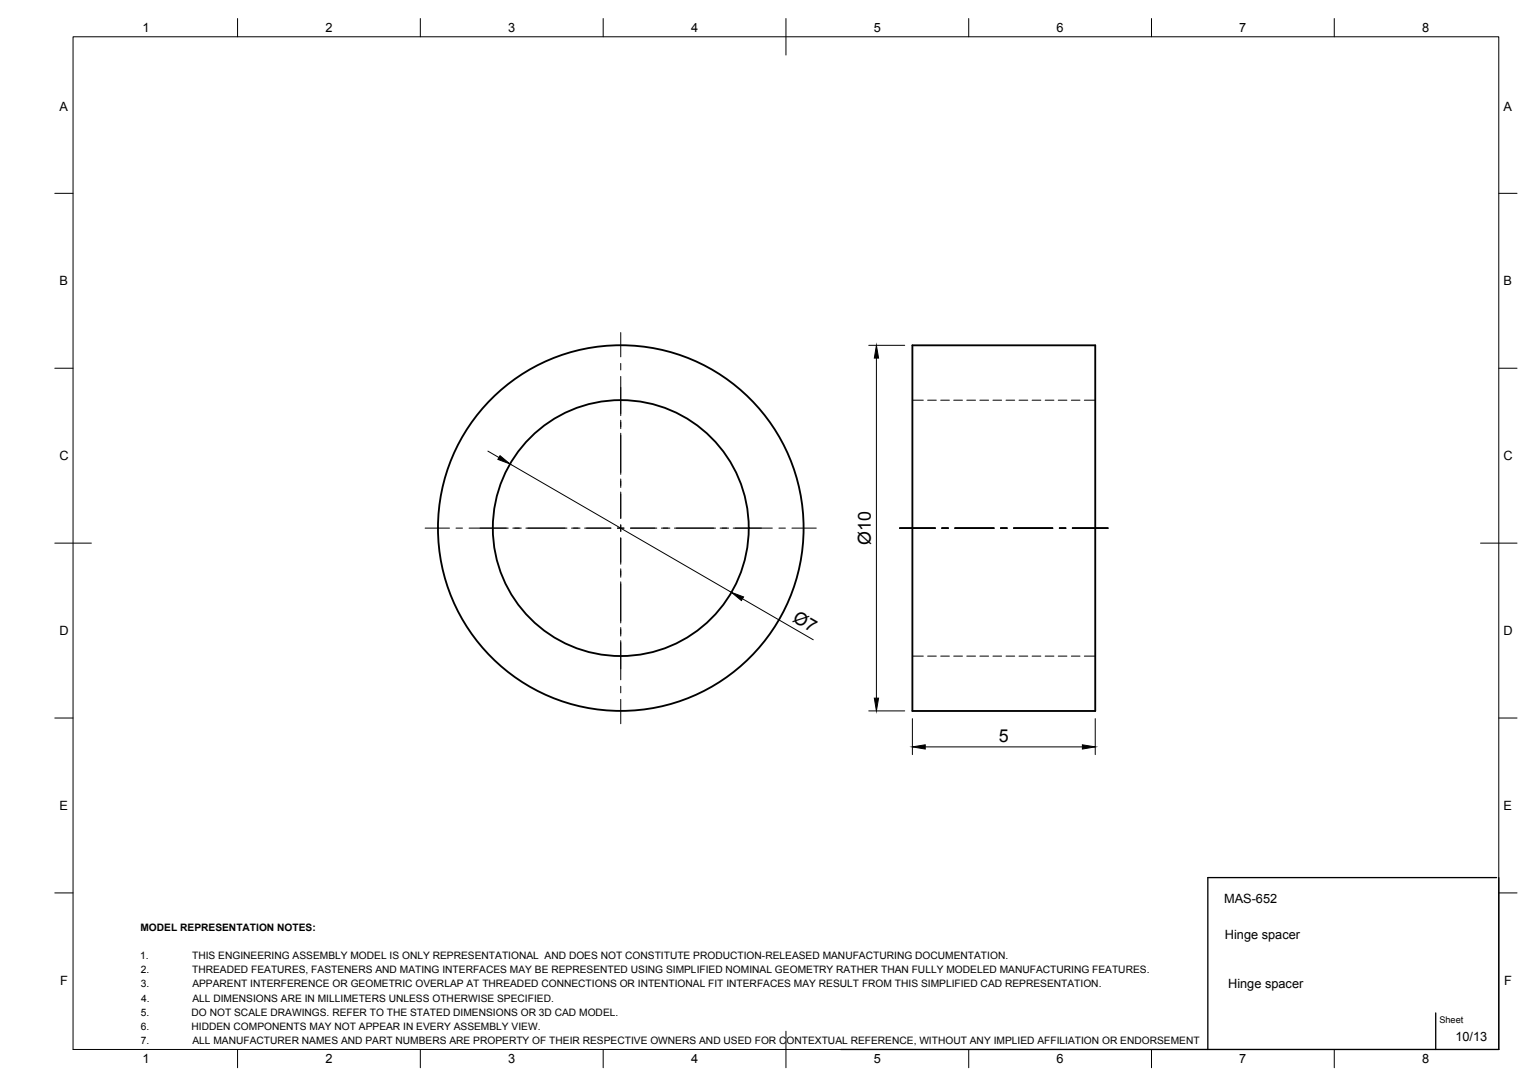
ISO-10303-21;
HEADER;
/* Generated by software containing ST-Developer
 * from STEP Tools, Inc. (www.steptools.com) 
 */

FILE_DESCRIPTION(
/* description */ ('Independent hinged machine back cover with retained hinge pins, perim
eter gasket and quarter-turn cam latch. Nominal cover 360 x 260 x 3 mm
, frame 430 x 300 x 20 mm. No guarding, structural or ingress rating a
ssigned.'),
/* implementation_level */ '2;1');

FILE_NAME(
/* name */ 'Hinge spacer.step',
/* time_stamp */ '2026-11-09T19:36:59-08:00',
/* author */ (''),
/* organization */ (''),
/* preprocessor_version */ 'ST-DEVELOPER v20.2',
/* originating_system */ 'Autodesk Translation Framework v15.17.0.0',
/* authorisation */ '');

FILE_SCHEMA (('AUTOMOTIVE_DESIGN { 1 0 10303 214 3 1 1 }'));
ENDSEC;

DATA;
#10=MECHANICAL_DESIGN_GEOMETRIC_PRESENTATION_REPRESENTATION('',(#211),#32627);
#175=SHAPE_REPRESENTATION_RELATIONSHIP('SRR','None',#32721,#193);
#193=ADVANCED_BREP_SHAPE_REPRESENTATION('',(#229),#32622);
#211=STYLED_ITEM('',(#32812),#229);
#229=MANIFOLD_SOLID_BREP('Body1',#8688);
#283=FACE_BOUND('',#1332,.T.);
#284=FACE_BOUND('',#1334,.T.);
#420=PLANE('',#9352);
#421=PLANE('',#9353);
#805=FACE_OUTER_BOUND('',#1329,.T.);
#806=FACE_OUTER_BOUND('',#1330,.T.);
#807=FACE_OUTER_BOUND('',#1331,.T.);
#808=FACE_OUTER_BOUND('',#1333,.T.);
#1329=EDGE_LOOP('',(#7239,#7240,#7241,#7242));
#1330=EDGE_LOOP('',(#7243,#7244,#7245,#7246));
#1331=EDGE_LOOP('',(#7247));
#1332=EDGE_LOOP('',(#7248));
#1333=EDGE_LOOP('',(#7249));
#1334=EDGE_LOOP('',(#7250));
#1559=CIRCLE('',#9347,3.5);
#1560=CIRCLE('',#9348,3.5);
#1561=CIRCLE('',#9350,5.);
#1562=CIRCLE('',#9351,5.);
#2589=LINE('',#26386,#3135);
#2590=LINE('',#26392,#3136);
#3135=VECTOR('',#10855,3.5);
#3136=VECTOR('',#10862,5.);
#3891=VERTEX_POINT('',#26383);
#3892=VERTEX_POINT('',#26385);
#3893=VERTEX_POINT('',#26389);
#3894=VERTEX_POINT('',#26391);
#5043=EDGE_CURVE('',#3891,#3891,#1559,.T.);
#5044=EDGE_CURVE('',#3891,#3892,#2589,.T.);
#5045=EDGE_CURVE('',#3892,#3892,#1560,.T.);
#5046=EDGE_CURVE('',#3893,#3893,#1561,.T.);
#5047=EDGE_CURVE('',#3893,#3894,#2590,.T.);
#5048=EDGE_CURVE('',#3894,#3894,#1562,.T.);
#7239=ORIENTED_EDGE('',*,*,#5043,.F.);
#7240=ORIENTED_EDGE('',*,*,#5044,.T.);
#7241=ORIENTED_EDGE('',*,*,#5045,.T.);
#7242=ORIENTED_EDGE('',*,*,#5044,.F.);
#7243=ORIENTED_EDGE('',*,*,#5046,.F.);
#7244=ORIENTED_EDGE('',*,*,#5047,.T.);
#7245=ORIENTED_EDGE('',*,*,#5048,.T.);
#7246=ORIENTED_EDGE('',*,*,#5047,.F.);
#7247=ORIENTED_EDGE('',*,*,#5046,.T.);
#7248=ORIENTED_EDGE('',*,*,#5043,.T.);
#7249=ORIENTED_EDGE('',*,*,#5048,.F.);
#7250=ORIENTED_EDGE('',*,*,#5045,.F.);
#8118=CYLINDRICAL_SURFACE('',#9346,3.5);
#8119=CYLINDRICAL_SURFACE('',#9349,5.);
#8553=ADVANCED_FACE('',(#805),#8118,.F.);
#8554=ADVANCED_FACE('',(#806),#8119,.T.);
#8555=ADVANCED_FACE('',(#807,#283),#420,.T.);
#8556=ADVANCED_FACE('',(#808,#284),#421,.F.);
#8688=CLOSED_SHELL('',(#8553,#8554,#8555,#8556));
#9345=AXIS2_PLACEMENT_3D('',#26381,#10849,#10850);
#9346=AXIS2_PLACEMENT_3D('',#26382,#10851,#10852);
#9347=AXIS2_PLACEMENT_3D('',#26384,#10853,#10854);
#9348=AXIS2_PLACEMENT_3D('',#26387,#10856,#10857);
#9349=AXIS2_PLACEMENT_3D('',#26388,#10858,#10859);
#9350=AXIS2_PLACEMENT_3D('',#26390,#10860,#10861);
#9351=AXIS2_PLACEMENT_3D('',#26393,#10863,#10864);
#9352=AXIS2_PLACEMENT_3D('',#26394,#10865,#10866);
#9353=AXIS2_PLACEMENT_3D('',#26395,#10867,#10868);
#10849=DIRECTION('axis',(0.,0.,1.));
#10850=DIRECTION('refdir',(1.,0.,0.));
#10851=DIRECTION('center_axis',(0.,0.,1.));
#10852=DIRECTION('ref_axis',(1.,0.,0.));
#10853=DIRECTION('center_axis',(0.,0.,-1.));
#10854=DIRECTION('ref_axis',(1.,0.,0.));
#10855=DIRECTION('',(0.,0.,-1.));
#10856=DIRECTION('center_axis',(0.,0.,-1.));
#10857=DIRECTION('ref_axis',(1.,0.,0.));
#10858=DIRECTION('center_axis',(0.,0.,1.));
#10859=DIRECTION('ref_axis',(1.,0.,0.));
#10860=DIRECTION('center_axis',(0.,0.,1.));
#10861=DIRECTION('ref_axis',(1.,0.,0.));
#10862=DIRECTION('',(0.,0.,-1.));
#10863=DIRECTION('center_axis',(0.,0.,1.));
#10864=DIRECTION('ref_axis',(1.,0.,0.));
#10865=DIRECTION('center_axis',(0.,0.,1.));
#10866=DIRECTION('ref_axis',(1.,0.,0.));
#10867=DIRECTION('center_axis',(0.,0.,1.));
#10868=DIRECTION('ref_axis',(1.,0.,0.));
#26381=CARTESIAN_POINT('',(0.,0.,0.));
#26382=CARTESIAN_POINT('Origin',(0.,0.,0.));
#26383=CARTESIAN_POINT('',(-3.5,-4.28626379701574E-16,5.));
#26384=CARTESIAN_POINT('Origin',(0.,0.,5.));
#26385=CARTESIAN_POINT('',(-3.5,-4.28626379701574E-16,0.));
#26386=CARTESIAN_POINT('',(-3.5,-4.28626379701574E-16,0.));
#26387=CARTESIAN_POINT('Origin',(0.,0.,0.));
#26388=CARTESIAN_POINT('Origin',(0.,0.,0.));
#26389=CARTESIAN_POINT('',(-5.,-6.12323399573677E-16,5.));
#26390=CARTESIAN_POINT('Origin',(0.,0.,5.));
#26391=CARTESIAN_POINT('',(-5.,-6.12323399573677E-16,0.));
#26392=CARTESIAN_POINT('',(-5.,-6.12323399573677E-16,0.));
#26393=CARTESIAN_POINT('Origin',(0.,0.,0.));
#26394=CARTESIAN_POINT('Origin',(0.,0.,5.));
#26395=CARTESIAN_POINT('Origin',(0.,0.,0.));
#32602=UNCERTAINTY_MEASURE_WITH_UNIT(LENGTH_MEASURE(0.01),#32628,
'DISTANCE_ACCURACY_VALUE',
'Maximum model space distance between geometric entities at asserted c
onnectivities');
#32607=UNCERTAINTY_MEASURE_WITH_UNIT(LENGTH_MEASURE(0.01),#32628,
'DISTANCE_ACCURACY_VALUE',
'Maximum model space distance between geometric entities at asserted c
onnectivities');
#32622=(
GEOMETRIC_REPRESENTATION_CONTEXT(3)
GLOBAL_UNCERTAINTY_ASSIGNED_CONTEXT((#32602))
GLOBAL_UNIT_ASSIGNED_CONTEXT((#32628,#32630,#32631))
REPRESENTATION_CONTEXT('','3D')
);
#32627=(
GEOMETRIC_REPRESENTATION_CONTEXT(3)
GLOBAL_UNCERTAINTY_ASSIGNED_CONTEXT((#32607))
GLOBAL_UNIT_ASSIGNED_CONTEXT((#32628,#32630,#32631))
REPRESENTATION_CONTEXT('','3D')
);
#32628=(
LENGTH_UNIT()
NAMED_UNIT(*)
SI_UNIT(.MILLI.,.METRE.)
);
#32630=(
NAMED_UNIT(*)
PLANE_ANGLE_UNIT()
SI_UNIT($,.RADIAN.)
);
#32631=(
NAMED_UNIT(*)
SI_UNIT($,.STERADIAN.)
SOLID_ANGLE_UNIT()
);
#32646=SHAPE_DEFINITION_REPRESENTATION(#32665,#32721);
#32665=PRODUCT_DEFINITION_SHAPE('',$,#32741);
#32721=SHAPE_REPRESENTATION('',(#9345),#32622);
#32726=PRODUCT_DEFINITION_CONTEXT('part definition',#32785,'design');
#32741=PRODUCT_DEFINITION('Hinge spacer','Hinge spacer',#32760,#32726);
#32760=PRODUCT_DEFINITION_FORMATION('',$,#32801);
#32785=APPLICATION_CONTEXT(
'Core Data for Automotive Mechanical Design Process');
#32786=PRODUCT_CONTEXT('part definition',#32785,'mechanical');
#32801=PRODUCT('Hinge spacer','Hinge spacer',$,(#32786));
#32812=PRESENTATION_STYLE_ASSIGNMENT((#32819));
#32819=SURFACE_STYLE_USAGE(.BOTH.,#32826);
#32826=SURFACE_SIDE_STYLE('',(#32833));
#32833=SURFACE_STYLE_FILL_AREA(#32840);
#32840=FILL_AREA_STYLE('Light gray',(#32847));
#32847=FILL_AREA_STYLE_COLOUR('Light gray',#32854);
#32854=COLOUR_RGB('Light gray',0.725490196078431,0.752941176470588,0.792156862745098);
ENDSEC;
END-ISO-10303-21;
